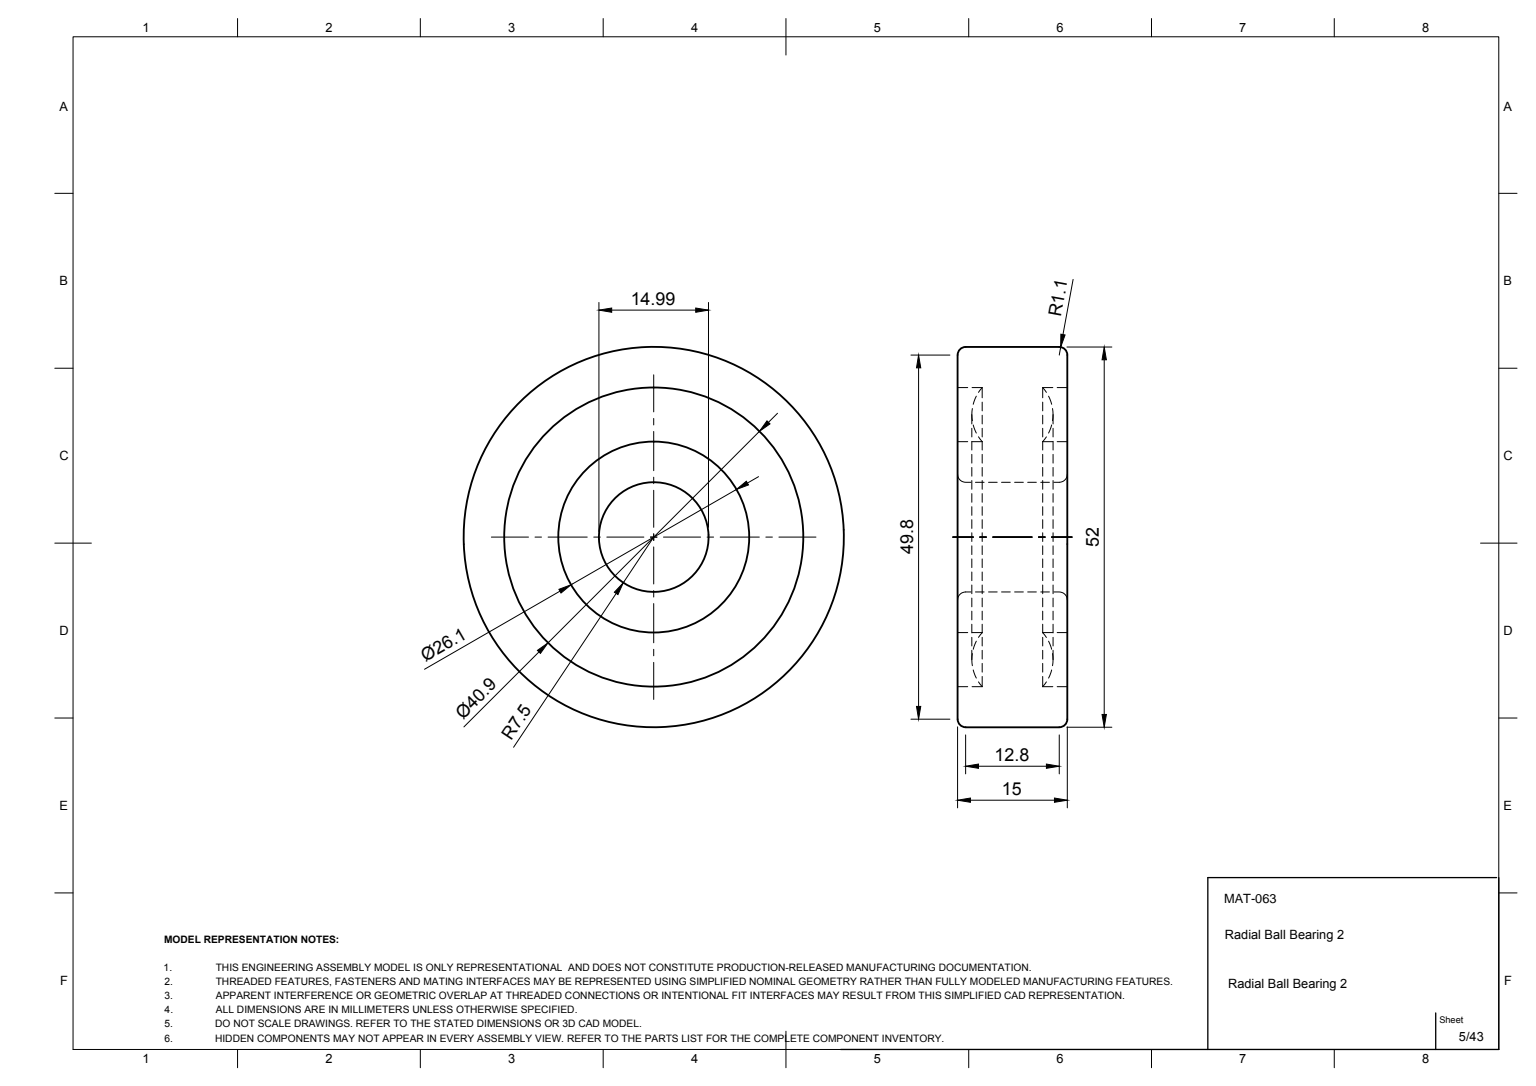
ISO-10303-21;
HEADER;
/* Generated by software containing ST-Developer
 * from STEP Tools, Inc. (www.steptools.com) 
 */

FILE_DESCRIPTION(
/* description */ (''),
/* implementation_level */ '2;1');

FILE_NAME(
/* name */ 'Radial Ball Bearing 2.step',
/* time_stamp */ '2026-10-24T09:43:01-07:00',
/* author */ (''),
/* organization */ (''),
/* preprocessor_version */ 'ST-DEVELOPER v20.2',
/* originating_system */ 'Autodesk Translation Framework v15.15.0.0',
/* authorisation */ '');

FILE_SCHEMA (('AUTOMOTIVE_DESIGN { 1 0 10303 214 3 1 1 }'));
ENDSEC;

DATA;
#10=MECHANICAL_DESIGN_GEOMETRIC_PRESENTATION_REPRESENTATION('',(#275),#11112);
#177=TOROIDAL_SURFACE('',#6521,0.0248999989285722,0.00110000131901909);
#178=TOROIDAL_SURFACE('',#6526,0.0248999989285722,0.00110000131901909);
#179=TOROIDAL_SURFACE('',#6534,0.0248999989285722,0.00110000131901911);
#180=TOROIDAL_SURFACE('',#6541,0.0248999989285722,0.00110000131901911);
#181=TOROIDAL_SURFACE('',#6545,0.01675,0.00555000054498457);
#182=TOROIDAL_SURFACE('',#6554,0.01675,0.00555000054498457);
#183=TOROIDAL_SURFACE('',#6563,0.00860000107142784,0.00110000131901912);
#184=TOROIDAL_SURFACE('',#6567,0.00860000107142784,0.00110000131901912);
#185=TOROIDAL_SURFACE('',#6575,0.00860000107142785,0.00110000131901912);
#186=TOROIDAL_SURFACE('',#6578,0.00860000107142785,0.00110000131901912);
#209=SHAPE_REPRESENTATION_RELATIONSHIP('SRR','None',#11232,#242);
#242=ADVANCED_BREP_SHAPE_REPRESENTATION('',(#308),#11077);
#275=STYLED_ITEM('',(#11425),#308);
#308=MANIFOLD_SOLID_BREP('Radial Ball Bearing 2',#6012);
#361=FACE_BOUND('',#1105,.T.);
#362=FACE_BOUND('',#1110,.T.);
#363=FACE_BOUND('',#1116,.T.);
#364=FACE_BOUND('',#1121,.T.);
#506=PLANE('',#6532);
#507=PLANE('',#6543);
#508=PLANE('',#6558);
#509=PLANE('',#6569);
#715=FACE_OUTER_BOUND('',#1101,.T.);
#716=FACE_OUTER_BOUND('',#1102,.T.);
#717=FACE_OUTER_BOUND('',#1103,.T.);
#718=FACE_OUTER_BOUND('',#1104,.T.);
#719=FACE_OUTER_BOUND('',#1106,.T.);
#720=FACE_OUTER_BOUND('',#1107,.T.);
#721=FACE_OUTER_BOUND('',#1108,.T.);
#722=FACE_OUTER_BOUND('',#1109,.T.);
#723=FACE_OUTER_BOUND('',#1111,.T.);
#724=FACE_OUTER_BOUND('',#1112,.T.);
#725=FACE_OUTER_BOUND('',#1113,.T.);
#726=FACE_OUTER_BOUND('',#1114,.T.);
#727=FACE_OUTER_BOUND('',#1115,.T.);
#728=FACE_OUTER_BOUND('',#1117,.T.);
#729=FACE_OUTER_BOUND('',#1118,.T.);
#730=FACE_OUTER_BOUND('',#1119,.T.);
#731=FACE_OUTER_BOUND('',#1120,.T.);
#732=FACE_OUTER_BOUND('',#1122,.T.);
#733=FACE_OUTER_BOUND('',#1123,.T.);
#734=FACE_OUTER_BOUND('',#1124,.T.);
#1101=EDGE_LOOP('',(#4133,#4134,#4135,#4136));
#1102=EDGE_LOOP('',(#4137,#4138,#4139,#4140));
#1103=EDGE_LOOP('',(#4141,#4142,#4143,#4144,#4145,#4146));
#1104=EDGE_LOOP('',(#4147,#4148));
#1105=EDGE_LOOP('',(#4149));
#1106=EDGE_LOOP('',(#4150,#4151,#4152,#4153));
#1107=EDGE_LOOP('',(#4154,#4155,#4156,#4157,#4158));
#1108=EDGE_LOOP('',(#4159,#4160,#4161,#4162));
#1109=EDGE_LOOP('',(#4163,#4164));
#1110=EDGE_LOOP('',(#4165));
#1111=EDGE_LOOP('',(#4166,#4167,#4168,#4169,#4170,#4171));
#1112=EDGE_LOOP('',(#4172,#4173,#4174,#4175,#4176));
#1113=EDGE_LOOP('',(#4177,#4178,#4179,#4180,#4181));
#1114=EDGE_LOOP('',(#4182,#4183,#4184,#4185,#4186,#4187));
#1115=EDGE_LOOP('',(#4188));
#1116=EDGE_LOOP('',(#4189,#4190));
#1117=EDGE_LOOP('',(#4191,#4192,#4193,#4194,#4195));
#1118=EDGE_LOOP('',(#4196,#4197,#4198,#4199));
#1119=EDGE_LOOP('',(#4200,#4201,#4202,#4203));
#1120=EDGE_LOOP('',(#4204));
#1121=EDGE_LOOP('',(#4205,#4206));
#1122=EDGE_LOOP('',(#4207,#4208,#4209,#4210,#4211,#4212));
#1123=EDGE_LOOP('',(#4213,#4214,#4215,#4216));
#1124=EDGE_LOOP('',(#4217,#4218,#4219,#4220));
#1580=LINE('',#9536,#1939);
#1581=LINE('',#9548,#1940);
#1582=LINE('',#9568,#1941);
#1583=LINE('',#9571,#1942);
#1584=LINE('',#9587,#1943);
#1585=LINE('',#9603,#1944);
#1939=VECTOR('',#7532,0.026);
#1940=VECTOR('',#7547,0.02045);
#1941=VECTOR('',#7574,0.02045);
#1942=VECTOR('',#7577,0.01305);
#1943=VECTOR('',#7598,0.01305);
#1944=VECTOR('',#7619,0.0075);
#2344=CIRCLE('',#6522,0.0248999997701383);
#2345=CIRCLE('',#6523,0.00110000131901909);
#2346=CIRCLE('',#6524,0.0260000002475909);
#2347=CIRCLE('',#6525,0.00110000131901909);
#2348=CIRCLE('',#6527,0.0248999997701383);
#2349=CIRCLE('',#6528,0.0260000002475909);
#2350=CIRCLE('',#6530,0.026);
#2351=CIRCLE('',#6531,0.026);
#2352=CIRCLE('',#6533,0.02045);
#2353=CIRCLE('',#6535,0.00110000131901911);
#2354=CIRCLE('',#6536,0.0248999997701383);
#2355=CIRCLE('',#6537,0.0011000013190191);
#2356=CIRCLE('',#6539,0.02045);
#2357=CIRCLE('',#6540,0.02045);
#2358=CIRCLE('',#6542,0.0248999997701383);
#2359=CIRCLE('',#6544,0.02045);
#2360=CIRCLE('',#6546,0.00555000054498457);
#2361=CIRCLE('',#6547,0.0130499999271107);
#2362=CIRCLE('',#6548,0.0130499999271107);
#2363=CIRCLE('',#6550,0.02045);
#2364=CIRCLE('',#6551,0.02045);
#2365=CIRCLE('',#6553,0.01305);
#2366=CIRCLE('',#6555,0.01305);
#2367=CIRCLE('',#6556,0.00555000054498457);
#2368=CIRCLE('',#6557,0.01305);
#2369=CIRCLE('',#6559,0.00860000022986177);
#2370=CIRCLE('',#6560,0.00860000022986177);
#2371=CIRCLE('',#6562,0.01305);
#2372=CIRCLE('',#6564,0.00110000131901912);
#2373=CIRCLE('',#6565,0.00749999975240907);
#2374=CIRCLE('',#6566,0.00110000131901912);
#2375=CIRCLE('',#6568,0.00749999975240873);
#2376=CIRCLE('',#6570,0.00860000022986177);
#2377=CIRCLE('',#6571,0.00860000022986177);
#2378=CIRCLE('',#6573,0.0075);
#2379=CIRCLE('',#6574,0.00749999975240873);
#2380=CIRCLE('',#6576,0.00110000131901912);
#2381=CIRCLE('',#6577,0.00110000131901912);
#2740=VERTEX_POINT('',#9520);
#2741=VERTEX_POINT('',#9521);
#2742=VERTEX_POINT('',#9523);
#2743=VERTEX_POINT('',#9525);
#2744=VERTEX_POINT('',#9532);
#2745=VERTEX_POINT('',#9533);
#2746=VERTEX_POINT('',#9538);
#2747=VERTEX_POINT('',#9541);
#2748=VERTEX_POINT('',#9543);
#2749=VERTEX_POINT('',#9547);
#2750=VERTEX_POINT('',#9549);
#2751=VERTEX_POINT('',#9555);
#2752=VERTEX_POINT('',#9558);
#2753=VERTEX_POINT('',#9560);
#2754=VERTEX_POINT('',#9564);
#2755=VERTEX_POINT('',#9565);
#2756=VERTEX_POINT('',#9570);
#2757=VERTEX_POINT('',#9574);
#2758=VERTEX_POINT('',#9575);
#2759=VERTEX_POINT('',#9580);
#2760=VERTEX_POINT('',#9581);
#2761=VERTEX_POINT('',#9585);
#2762=VERTEX_POINT('',#9589);
#2763=VERTEX_POINT('',#9591);
#2764=VERTEX_POINT('',#9597);
#2765=VERTEX_POINT('',#9598);
#2766=VERTEX_POINT('',#9602);
#2767=VERTEX_POINT('',#9604);
#3270=EDGE_CURVE('',#2740,#2741,#2344,.T.);
#3271=EDGE_CURVE('',#2741,#2742,#2345,.T.);
#3272=EDGE_CURVE('',#2742,#2743,#2346,.F.);
#3273=EDGE_CURVE('',#2743,#2740,#2347,.T.);
#3274=EDGE_CURVE('',#2741,#2740,#2348,.T.);
#3275=EDGE_CURVE('',#2743,#2742,#2349,.T.);
#3276=EDGE_CURVE('',#2744,#2745,#2350,.F.);
#3277=EDGE_CURVE('',#2745,#2744,#2351,.F.);
#3278=EDGE_CURVE('',#2744,#2742,#1580,.T.);
#3279=EDGE_CURVE('',#2746,#2746,#2352,.T.);
#3280=EDGE_CURVE('',#2744,#2747,#2353,.T.);
#3281=EDGE_CURVE('',#2747,#2748,#2354,.F.);
#3282=EDGE_CURVE('',#2748,#2745,#2355,.T.);
#3283=EDGE_CURVE('',#2746,#2749,#1581,.T.);
#3284=EDGE_CURVE('',#2750,#2749,#2356,.F.);
#3285=EDGE_CURVE('',#2749,#2750,#2357,.F.);
#3286=EDGE_CURVE('',#2748,#2747,#2358,.F.);
#3287=EDGE_CURVE('',#2751,#2751,#2359,.F.);
#3288=EDGE_CURVE('',#2750,#2752,#2360,.T.);
#3289=EDGE_CURVE('',#2752,#2753,#2361,.T.);
#3290=EDGE_CURVE('',#2753,#2752,#2362,.T.);
#3291=EDGE_CURVE('',#2754,#2755,#2363,.F.);
#3292=EDGE_CURVE('',#2755,#2754,#2364,.F.);
#3293=EDGE_CURVE('',#2755,#2751,#1582,.T.);
#3294=EDGE_CURVE('',#2753,#2756,#1583,.T.);
#3295=EDGE_CURVE('',#2756,#2756,#2365,.T.);
#3296=EDGE_CURVE('',#2757,#2758,#2366,.T.);
#3297=EDGE_CURVE('',#2758,#2754,#2367,.T.);
#3298=EDGE_CURVE('',#2758,#2757,#2368,.T.);
#3299=EDGE_CURVE('',#2759,#2760,#2369,.T.);
#3300=EDGE_CURVE('',#2760,#2759,#2370,.T.);
#3301=EDGE_CURVE('',#2761,#2761,#2371,.F.);
#3302=EDGE_CURVE('',#2761,#2757,#1584,.T.);
#3303=EDGE_CURVE('',#2760,#2762,#2372,.T.);
#3304=EDGE_CURVE('',#2762,#2763,#2373,.T.);
#3305=EDGE_CURVE('',#2763,#2759,#2374,.T.);
#3306=EDGE_CURVE('',#2763,#2762,#2375,.T.);
#3307=EDGE_CURVE('',#2764,#2765,#2376,.F.);
#3308=EDGE_CURVE('',#2765,#2764,#2377,.F.);
#3309=EDGE_CURVE('',#2762,#2766,#1585,.T.);
#3310=EDGE_CURVE('',#2767,#2766,#2378,.F.);
#3311=EDGE_CURVE('',#2766,#2767,#2379,.F.);
#3312=EDGE_CURVE('',#2766,#2764,#2380,.T.);
#3313=EDGE_CURVE('',#2765,#2767,#2381,.T.);
#4133=ORIENTED_EDGE('',*,*,#3270,.T.);
#4134=ORIENTED_EDGE('',*,*,#3271,.T.);
#4135=ORIENTED_EDGE('',*,*,#3272,.T.);
#4136=ORIENTED_EDGE('',*,*,#3273,.T.);
#4137=ORIENTED_EDGE('',*,*,#3271,.F.);
#4138=ORIENTED_EDGE('',*,*,#3274,.T.);
#4139=ORIENTED_EDGE('',*,*,#3273,.F.);
#4140=ORIENTED_EDGE('',*,*,#3275,.T.);
#4141=ORIENTED_EDGE('',*,*,#3276,.T.);
#4142=ORIENTED_EDGE('',*,*,#3277,.T.);
#4143=ORIENTED_EDGE('',*,*,#3278,.T.);
#4144=ORIENTED_EDGE('',*,*,#3275,.F.);
#4145=ORIENTED_EDGE('',*,*,#3272,.F.);
#4146=ORIENTED_EDGE('',*,*,#3278,.F.);
#4147=ORIENTED_EDGE('',*,*,#3270,.F.);
#4148=ORIENTED_EDGE('',*,*,#3274,.F.);
#4149=ORIENTED_EDGE('',*,*,#3279,.T.);
#4150=ORIENTED_EDGE('',*,*,#3276,.F.);
#4151=ORIENTED_EDGE('',*,*,#3280,.T.);
#4152=ORIENTED_EDGE('',*,*,#3281,.T.);
#4153=ORIENTED_EDGE('',*,*,#3282,.T.);
#4154=ORIENTED_EDGE('',*,*,#3279,.F.);
#4155=ORIENTED_EDGE('',*,*,#3283,.T.);
#4156=ORIENTED_EDGE('',*,*,#3284,.F.);
#4157=ORIENTED_EDGE('',*,*,#3285,.F.);
#4158=ORIENTED_EDGE('',*,*,#3283,.F.);
#4159=ORIENTED_EDGE('',*,*,#3280,.F.);
#4160=ORIENTED_EDGE('',*,*,#3277,.F.);
#4161=ORIENTED_EDGE('',*,*,#3282,.F.);
#4162=ORIENTED_EDGE('',*,*,#3286,.T.);
#4163=ORIENTED_EDGE('',*,*,#3281,.F.);
#4164=ORIENTED_EDGE('',*,*,#3286,.F.);
#4165=ORIENTED_EDGE('',*,*,#3287,.T.);
#4166=ORIENTED_EDGE('',*,*,#3285,.T.);
#4167=ORIENTED_EDGE('',*,*,#3288,.T.);
#4168=ORIENTED_EDGE('',*,*,#3289,.T.);
#4169=ORIENTED_EDGE('',*,*,#3290,.T.);
#4170=ORIENTED_EDGE('',*,*,#3288,.F.);
#4171=ORIENTED_EDGE('',*,*,#3284,.T.);
#4172=ORIENTED_EDGE('',*,*,#3291,.F.);
#4173=ORIENTED_EDGE('',*,*,#3292,.F.);
#4174=ORIENTED_EDGE('',*,*,#3293,.T.);
#4175=ORIENTED_EDGE('',*,*,#3287,.F.);
#4176=ORIENTED_EDGE('',*,*,#3293,.F.);
#4177=ORIENTED_EDGE('',*,*,#3290,.F.);
#4178=ORIENTED_EDGE('',*,*,#3294,.T.);
#4179=ORIENTED_EDGE('',*,*,#3295,.T.);
#4180=ORIENTED_EDGE('',*,*,#3294,.F.);
#4181=ORIENTED_EDGE('',*,*,#3289,.F.);
#4182=ORIENTED_EDGE('',*,*,#3296,.T.);
#4183=ORIENTED_EDGE('',*,*,#3297,.T.);
#4184=ORIENTED_EDGE('',*,*,#3291,.T.);
#4185=ORIENTED_EDGE('',*,*,#3292,.T.);
#4186=ORIENTED_EDGE('',*,*,#3297,.F.);
#4187=ORIENTED_EDGE('',*,*,#3298,.T.);
#4188=ORIENTED_EDGE('',*,*,#3295,.F.);
#4189=ORIENTED_EDGE('',*,*,#3299,.T.);
#4190=ORIENTED_EDGE('',*,*,#3300,.T.);
#4191=ORIENTED_EDGE('',*,*,#3301,.T.);
#4192=ORIENTED_EDGE('',*,*,#3302,.T.);
#4193=ORIENTED_EDGE('',*,*,#3298,.F.);
#4194=ORIENTED_EDGE('',*,*,#3296,.F.);
#4195=ORIENTED_EDGE('',*,*,#3302,.F.);
#4196=ORIENTED_EDGE('',*,*,#3303,.T.);
#4197=ORIENTED_EDGE('',*,*,#3304,.T.);
#4198=ORIENTED_EDGE('',*,*,#3305,.T.);
#4199=ORIENTED_EDGE('',*,*,#3300,.F.);
#4200=ORIENTED_EDGE('',*,*,#3306,.T.);
#4201=ORIENTED_EDGE('',*,*,#3303,.F.);
#4202=ORIENTED_EDGE('',*,*,#3299,.F.);
#4203=ORIENTED_EDGE('',*,*,#3305,.F.);
#4204=ORIENTED_EDGE('',*,*,#3301,.F.);
#4205=ORIENTED_EDGE('',*,*,#3307,.T.);
#4206=ORIENTED_EDGE('',*,*,#3308,.T.);
#4207=ORIENTED_EDGE('',*,*,#3304,.F.);
#4208=ORIENTED_EDGE('',*,*,#3309,.T.);
#4209=ORIENTED_EDGE('',*,*,#3310,.F.);
#4210=ORIENTED_EDGE('',*,*,#3311,.F.);
#4211=ORIENTED_EDGE('',*,*,#3309,.F.);
#4212=ORIENTED_EDGE('',*,*,#3306,.F.);
#4213=ORIENTED_EDGE('',*,*,#3312,.T.);
#4214=ORIENTED_EDGE('',*,*,#3308,.F.);
#4215=ORIENTED_EDGE('',*,*,#3313,.T.);
#4216=ORIENTED_EDGE('',*,*,#3310,.T.);
#4217=ORIENTED_EDGE('',*,*,#3307,.F.);
#4218=ORIENTED_EDGE('',*,*,#3312,.F.);
#4219=ORIENTED_EDGE('',*,*,#3311,.T.);
#4220=ORIENTED_EDGE('',*,*,#3313,.F.);
#5519=CYLINDRICAL_SURFACE('',#6529,0.026);
#5520=CYLINDRICAL_SURFACE('',#6538,0.02045);
#5521=CYLINDRICAL_SURFACE('',#6549,0.02045);
#5522=CYLINDRICAL_SURFACE('',#6552,0.01305);
#5523=CYLINDRICAL_SURFACE('',#6561,0.01305);
#5524=CYLINDRICAL_SURFACE('',#6572,0.0075);
#5688=ADVANCED_FACE('',(#715),#177,.T.);
#5689=ADVANCED_FACE('',(#716),#178,.T.);
#5690=ADVANCED_FACE('',(#717),#5519,.T.);
#5691=ADVANCED_FACE('',(#718,#361),#506,.T.);
#5692=ADVANCED_FACE('',(#719),#179,.T.);
#5693=ADVANCED_FACE('',(#720),#5520,.F.);
#5694=ADVANCED_FACE('',(#721),#180,.T.);
#5695=ADVANCED_FACE('',(#722,#362),#507,.T.);
#5696=ADVANCED_FACE('',(#723),#181,.T.);
#5697=ADVANCED_FACE('',(#724),#5521,.F.);
#5698=ADVANCED_FACE('',(#725),#5522,.T.);
#5699=ADVANCED_FACE('',(#726),#182,.T.);
#5700=ADVANCED_FACE('',(#727,#363),#508,.T.);
#5701=ADVANCED_FACE('',(#728),#5523,.T.);
#5702=ADVANCED_FACE('',(#729),#183,.T.);
#5703=ADVANCED_FACE('',(#730),#184,.T.);
#5704=ADVANCED_FACE('',(#731,#364),#509,.T.);
#5705=ADVANCED_FACE('',(#732),#5524,.F.);
#5706=ADVANCED_FACE('',(#733),#185,.T.);
#5707=ADVANCED_FACE('',(#734),#186,.T.);
#6012=CLOSED_SHELL('',(#5688,#5689,#5690,#5691,#5692,#5693,#5694,#5695,
#5696,#5697,#5698,#5699,#5700,#5701,#5702,#5703,#5704,#5705,#5706,#5707));
#6520=AXIS2_PLACEMENT_3D('',#9518,#7508,#7509);
#6521=AXIS2_PLACEMENT_3D('',#9519,#7510,#7511);
#6522=AXIS2_PLACEMENT_3D('',#9522,#7512,#7513);
#6523=AXIS2_PLACEMENT_3D('',#9524,#7514,#7515);
#6524=AXIS2_PLACEMENT_3D('',#9526,#7516,#7517);
#6525=AXIS2_PLACEMENT_3D('',#9527,#7518,#7519);
#6526=AXIS2_PLACEMENT_3D('',#9528,#7520,#7521);
#6527=AXIS2_PLACEMENT_3D('',#9529,#7522,#7523);
#6528=AXIS2_PLACEMENT_3D('',#9530,#7524,#7525);
#6529=AXIS2_PLACEMENT_3D('',#9531,#7526,#7527);
#6530=AXIS2_PLACEMENT_3D('',#9534,#7528,#7529);
#6531=AXIS2_PLACEMENT_3D('',#9535,#7530,#7531);
#6532=AXIS2_PLACEMENT_3D('',#9537,#7533,#7534);
#6533=AXIS2_PLACEMENT_3D('',#9539,#7535,#7536);
#6534=AXIS2_PLACEMENT_3D('',#9540,#7537,#7538);
#6535=AXIS2_PLACEMENT_3D('',#9542,#7539,#7540);
#6536=AXIS2_PLACEMENT_3D('',#9544,#7541,#7542);
#6537=AXIS2_PLACEMENT_3D('',#9545,#7543,#7544);
#6538=AXIS2_PLACEMENT_3D('',#9546,#7545,#7546);
#6539=AXIS2_PLACEMENT_3D('',#9550,#7548,#7549);
#6540=AXIS2_PLACEMENT_3D('',#9551,#7550,#7551);
#6541=AXIS2_PLACEMENT_3D('',#9552,#7552,#7553);
#6542=AXIS2_PLACEMENT_3D('',#9553,#7554,#7555);
#6543=AXIS2_PLACEMENT_3D('',#9554,#7556,#7557);
#6544=AXIS2_PLACEMENT_3D('',#9556,#7558,#7559);
#6545=AXIS2_PLACEMENT_3D('',#9557,#7560,#7561);
#6546=AXIS2_PLACEMENT_3D('',#9559,#7562,#7563);
#6547=AXIS2_PLACEMENT_3D('',#9561,#7564,#7565);
#6548=AXIS2_PLACEMENT_3D('',#9562,#7566,#7567);
#6549=AXIS2_PLACEMENT_3D('',#9563,#7568,#7569);
#6550=AXIS2_PLACEMENT_3D('',#9566,#7570,#7571);
#6551=AXIS2_PLACEMENT_3D('',#9567,#7572,#7573);
#6552=AXIS2_PLACEMENT_3D('',#9569,#7575,#7576);
#6553=AXIS2_PLACEMENT_3D('',#9572,#7578,#7579);
#6554=AXIS2_PLACEMENT_3D('',#9573,#7580,#7581);
#6555=AXIS2_PLACEMENT_3D('',#9576,#7582,#7583);
#6556=AXIS2_PLACEMENT_3D('',#9577,#7584,#7585);
#6557=AXIS2_PLACEMENT_3D('',#9578,#7586,#7587);
#6558=AXIS2_PLACEMENT_3D('',#9579,#7588,#7589);
#6559=AXIS2_PLACEMENT_3D('',#9582,#7590,#7591);
#6560=AXIS2_PLACEMENT_3D('',#9583,#7592,#7593);
#6561=AXIS2_PLACEMENT_3D('',#9584,#7594,#7595);
#6562=AXIS2_PLACEMENT_3D('',#9586,#7596,#7597);
#6563=AXIS2_PLACEMENT_3D('',#9588,#7599,#7600);
#6564=AXIS2_PLACEMENT_3D('',#9590,#7601,#7602);
#6565=AXIS2_PLACEMENT_3D('',#9592,#7603,#7604);
#6566=AXIS2_PLACEMENT_3D('',#9593,#7605,#7606);
#6567=AXIS2_PLACEMENT_3D('',#9594,#7607,#7608);
#6568=AXIS2_PLACEMENT_3D('',#9595,#7609,#7610);
#6569=AXIS2_PLACEMENT_3D('',#9596,#7611,#7612);
#6570=AXIS2_PLACEMENT_3D('',#9599,#7613,#7614);
#6571=AXIS2_PLACEMENT_3D('',#9600,#7615,#7616);
#6572=AXIS2_PLACEMENT_3D('',#9601,#7617,#7618);
#6573=AXIS2_PLACEMENT_3D('',#9605,#7620,#7621);
#6574=AXIS2_PLACEMENT_3D('',#9606,#7622,#7623);
#6575=AXIS2_PLACEMENT_3D('',#9607,#7624,#7625);
#6576=AXIS2_PLACEMENT_3D('',#9608,#7626,#7627);
#6577=AXIS2_PLACEMENT_3D('',#9609,#7628,#7629);
#6578=AXIS2_PLACEMENT_3D('',#9610,#7630,#7631);
#7508=DIRECTION('axis',(0.,0.,1.));
#7509=DIRECTION('refdir',(1.,0.,0.));
#7510=DIRECTION('center_axis',(1.,4.17203717831812E-9,1.01277540341552E-17));
#7511=DIRECTION('ref_axis',(-4.1720371751696E-9,1.,0.));
#7512=DIRECTION('center_axis',(1.,4.17203717831812E-9,1.01277540341552E-17));
#7513=DIRECTION('ref_axis',(-4.17203717831812E-9,1.,-1.69634196247466E-42));
#7514=DIRECTION('center_axis',(8.36866394062756E-10,1.,-8.36884415538179E-10));
#7515=DIRECTION('ref_axis',(-7.96162761077703E-7,8.36885081819775E-10,0.999999999999683));
#7516=DIRECTION('center_axis',(1.,4.17203717831812E-9,1.01277540341552E-17));
#7517=DIRECTION('ref_axis',(-4.17203717831812E-9,1.,-1.69634196247466E-42));
#7518=DIRECTION('center_axis',(8.36869948186391E-10,1.,8.36891441629708E-10));
#7519=DIRECTION('ref_axis',(-0.999999999999707,8.36870588457614E-10,-7.65059166582913E-7));
#7520=DIRECTION('center_axis',(1.,-4.17203708245403E-9,6.73890284431642E-18));
#7521=DIRECTION('ref_axis',(-4.1720370750894E-9,-1.,5.66553889764798E-16));
#7522=DIRECTION('center_axis',(1.,-4.17203708245403E-9,6.73890284431642E-18));
#7523=DIRECTION('ref_axis',(4.17203708245403E-9,1.,-1.23465054354127E-43));
#7524=DIRECTION('center_axis',(-1.,4.17203697154146E-9,4.27849718847752E-19));
#7525=DIRECTION('ref_axis',(-4.27008851558771E-17,-5.34839554841822E-9,
1.));
#7526=DIRECTION('center_axis',(1.,0.,-3.33600668457079E-17));
#7527=DIRECTION('ref_axis',(-3.33600668457079E-17,0.,-1.));
#7528=DIRECTION('center_axis',(1.,0.,-3.33600668457079E-17));
#7529=DIRECTION('ref_axis',(-3.33600668457079E-17,0.,-1.));
#7530=DIRECTION('center_axis',(1.,0.,0.));
#7531=DIRECTION('ref_axis',(0.,-4.64793894161955E-10,-1.));
#7532=DIRECTION('',(-1.,0.,3.33600668457079E-17));
#7533=DIRECTION('center_axis',(-1.,1.53144334479515E-17,1.9842828066192E-17));
#7534=DIRECTION('ref_axis',(1.9842828066192E-17,0.,1.));
#7535=DIRECTION('center_axis',(1.,0.,0.));
#7536=DIRECTION('ref_axis',(0.,0.,-1.));
#7537=DIRECTION('center_axis',(1.,-4.17203727418451E-9,-1.07069540457721E-17));
#7538=DIRECTION('ref_axis',(4.1720372752498E-9,1.,0.));
#7539=DIRECTION('center_axis',(-8.36866342496331E-10,1.,-8.36883936494317E-10));
#7540=DIRECTION('ref_axis',(0.999999999999707,8.36866982761818E-10,7.65059174657239E-7));
#7541=DIRECTION('center_axis',(1.,-4.17203727418451E-9,-1.07069540457721E-17));
#7542=DIRECTION('ref_axis',(4.17203727418451E-9,1.,1.45967462857766E-42));
#7543=DIRECTION('center_axis',(-8.36844869453255E-10,1.,8.36865935422119E-10));
#7544=DIRECTION('ref_axis',(9.00645352209864E-7,8.36866689122222E-10,-0.999999999999595));
#7545=DIRECTION('center_axis',(1.,0.,0.));
#7546=DIRECTION('ref_axis',(0.,0.,-1.));
#7547=DIRECTION('',(1.,0.,0.));
#7548=DIRECTION('center_axis',(1.,0.,0.));
#7549=DIRECTION('ref_axis',(0.,-4.29586394988857E-10,-1.));
#7550=DIRECTION('center_axis',(1.,0.,0.));
#7551=DIRECTION('ref_axis',(0.,-4.29586394988857E-10,-1.));
#7552=DIRECTION('center_axis',(1.,4.17203725971588E-9,2.0031116033889E-18));
#7553=DIRECTION('ref_axis',(4.1720372752498E-9,-1.,5.66553889764798E-16));
#7554=DIRECTION('center_axis',(1.,4.17203725971588E-9,2.0031116033889E-18));
#7555=DIRECTION('ref_axis',(-4.17203725971588E-9,1.,5.39459847610519E-43));
#7556=DIRECTION('center_axis',(1.,1.53144334479515E-17,-1.9842828066192E-17));
#7557=DIRECTION('ref_axis',(-1.9842828066192E-17,0.,-1.));
#7558=DIRECTION('center_axis',(1.,0.,0.));
#7559=DIRECTION('ref_axis',(0.,0.,-1.));
#7560=DIRECTION('center_axis',(1.,6.36556116938371E-17,1.00386354793954E-17));
#7561=DIRECTION('ref_axis',(-6.3655612933414E-17,1.,0.));
#7562=DIRECTION('center_axis',(1.00386354793954E-17,1.22464679914735E-16,
-1.));
#7563=DIRECTION('ref_axis',(6.36556105223495E-17,-1.,-1.22464679914735E-16));
#7564=DIRECTION('center_axis',(1.,1.35504238326755E-16,2.34999225611352E-17));
#7565=DIRECTION('ref_axis',(-1.35504238326755E-16,1.,1.40763492406121E-49));
#7566=DIRECTION('center_axis',(1.,1.35504238326755E-16,2.34999225611352E-17));
#7567=DIRECTION('ref_axis',(-1.35504238326755E-16,1.,1.40763492406121E-49));
#7568=DIRECTION('center_axis',(1.,0.,0.));
#7569=DIRECTION('ref_axis',(0.,0.,-1.));
#7570=DIRECTION('center_axis',(-1.,0.,0.));
#7571=DIRECTION('ref_axis',(0.,-6.60206605267583E-10,1.));
#7572=DIRECTION('center_axis',(-1.,0.,0.));
#7573=DIRECTION('ref_axis',(0.,-6.60206605267583E-10,1.));
#7574=DIRECTION('',(1.,0.,0.));
#7575=DIRECTION('center_axis',(1.,0.,0.));
#7576=DIRECTION('ref_axis',(0.,0.,-1.));
#7577=DIRECTION('',(-1.,0.,0.));
#7578=DIRECTION('center_axis',(1.,0.,0.));
#7579=DIRECTION('ref_axis',(0.,0.,-1.));
#7580=DIRECTION('center_axis',(1.,1.18552772674719E-16,-1.97711088800387E-17));
#7581=DIRECTION('ref_axis',(-1.18552772074394E-16,1.,0.));
#7582=DIRECTION('center_axis',(-1.,0.,0.));
#7583=DIRECTION('ref_axis',(0.,-2.05103586755523E-10,1.));
#7584=DIRECTION('center_axis',(-1.97711088800387E-17,1.22464679914735E-16,
-1.));
#7585=DIRECTION('ref_axis',(1.18552771796194E-16,-1.,-1.22464679914735E-16));
#7586=DIRECTION('center_axis',(-1.,0.,0.));
#7587=DIRECTION('ref_axis',(0.,-2.05103586755523E-10,1.));
#7588=DIRECTION('center_axis',(-1.,2.92206431305708E-17,3.78610282642285E-17));
#7589=DIRECTION('ref_axis',(3.78610282642285E-17,0.,1.));
#7590=DIRECTION('center_axis',(1.,1.20795004338275E-8,6.525328094131E-17));
#7591=DIRECTION('ref_axis',(-1.20795004338275E-8,1.,4.44135209129409E-41));
#7592=DIRECTION('center_axis',(1.,-1.20794999078492E-8,-6.65136044666218E-17));
#7593=DIRECTION('ref_axis',(1.20794999078492E-8,1.,-3.20659696454606E-41));
#7594=DIRECTION('center_axis',(1.,0.,0.));
#7595=DIRECTION('ref_axis',(0.,0.,-1.));
#7596=DIRECTION('center_axis',(1.,0.,0.));
#7597=DIRECTION('ref_axis',(0.,0.,-1.));
#7598=DIRECTION('',(-1.,0.,0.));
#7599=DIRECTION('center_axis',(1.,-1.20794999078492E-8,-6.65136044666218E-17));
#7600=DIRECTION('ref_axis',(-1.20794999243885E-8,-1.,-5.21792575105832E-12));
#7601=DIRECTION('center_axis',(-3.90112644891662E-10,-1.,-3.90117034748036E-10));
#7602=DIRECTION('ref_axis',(-7.96162782272821E-7,3.90117345341081E-10,-0.999999999999683));
#7603=DIRECTION('center_axis',(1.,-1.20794992145421E-8,-4.8381018443521E-19));
#7604=DIRECTION('ref_axis',(1.48029741503464E-16,1.78300800621899E-8,-1.));
#7605=DIRECTION('center_axis',(-3.90083830404282E-10,-1.,3.90119162273478E-10));
#7606=DIRECTION('ref_axis',(-0.999999999999707,3.90084128868405E-10,7.65059156489968E-7));
#7607=DIRECTION('center_axis',(1.,1.20795004338275E-8,6.525328094131E-17));
#7608=DIRECTION('ref_axis',(-1.20795004609008E-8,1.,0.));
#7609=DIRECTION('center_axis',(1.,1.20795004338275E-8,6.525328094131E-17));
#7610=DIRECTION('ref_axis',(-1.20795004338275E-8,1.,4.44135209129409E-41));
#7611=DIRECTION('center_axis',(1.,2.92206431305708E-17,-3.78610282642285E-17));
#7612=DIRECTION('ref_axis',(-3.78610282642285E-17,0.,-1.));
#7613=DIRECTION('center_axis',(1.,-1.20794999071527E-8,2.28224857621035E-17));
#7614=DIRECTION('ref_axis',(1.20794999071527E-8,1.,-1.89856639006012E-41));
#7615=DIRECTION('center_axis',(1.,1.20794999172425E-8,-1.59545740616835E-17));
#7616=DIRECTION('ref_axis',(-1.20794999172425E-8,1.,2.99570552288603E-42));
#7617=DIRECTION('center_axis',(1.,0.,-1.15648231731787E-16));
#7618=DIRECTION('ref_axis',(-1.15648231731787E-16,0.,-1.));
#7619=DIRECTION('',(1.,0.,-1.15648231731787E-16));
#7620=DIRECTION('center_axis',(1.,0.,0.));
#7621=DIRECTION('ref_axis',(0.,-4.29586131949163E-10,-1.));
#7622=DIRECTION('center_axis',(1.,-1.20794999071527E-8,2.28224857621035E-17));
#7623=DIRECTION('ref_axis',(1.20794999071527E-8,1.,-1.89856639006012E-41));
#7624=DIRECTION('center_axis',(1.,1.20794999172425E-8,-1.59545740616835E-17));
#7625=DIRECTION('ref_axis',(1.20794999243885E-8,-1.,-8.2319592183107E-12));
#7626=DIRECTION('center_axis',(3.9010897446429E-10,-1.,-3.90108144056802E-10));
#7627=DIRECTION('ref_axis',(0.999999999999707,3.90109272919983E-10,-7.65059154471383E-7));
#7628=DIRECTION('center_axis',(3.90083837031876E-10,-1.,3.90119162425402E-10));
#7629=DIRECTION('ref_axis',(7.96162783282112E-7,3.90119472995512E-10,0.999999999999683));
#7630=DIRECTION('center_axis',(1.,-1.20794999071527E-8,2.28224857621035E-17));
#7631=DIRECTION('ref_axis',(1.20794999243885E-8,1.,0.));
#9518=CARTESIAN_POINT('',(0.,0.,0.));
#9519=CARTESIAN_POINT('Origin',(-0.00639999889435817,-1.33725586897056E-10,
-2.60202312123977E-18));
#9520=CARTESIAN_POINT('',(-0.00750000021337694,-2.62982038223811E-17,-0.0248999997701383));
#9521=CARTESIAN_POINT('',(-0.00750000021337694,-9.33158505355009E-18,0.0248999997701383));
#9522=CARTESIAN_POINT('Origin',(-0.00750000021337694,-1.38314833296201E-10,
-2.61316366403604E-18));
#9523=CARTESIAN_POINT('',(-0.00639999976976533,-1.58005919577827E-12,0.0260000002475909));
#9524=CARTESIAN_POINT('Origin',(-0.00639999889435817,-9.20581548326642E-13,
0.0248999989285722));
#9525=CARTESIAN_POINT('',(-0.00639999976976533,-3.35121902792442E-17,-0.0260000002475909));
#9526=CARTESIAN_POINT('Origin',(-0.00639999977013826,-1.33725590550843E-10,
-2.60202313010945E-18));
#9527=CARTESIAN_POINT('Origin',(-0.00639999889435817,-9.20629689158185E-13,
-0.0248999989285722));
#9528=CARTESIAN_POINT('Origin',(-0.00639999889435817,1.33725588194013E-10,
-2.25687613815873E-19));
#9529=CARTESIAN_POINT('Origin',(-0.00750000021337694,1.38314834487708E-10,
-2.3310041583336E-19));
#9530=CARTESIAN_POINT('Origin',(-0.00639999977013826,1.3372558821988E-10,
4.44089209850063E-18));
#9531=CARTESIAN_POINT('Origin',(-0.0206375,0.,-4.33144407778805E-52));
#9532=CARTESIAN_POINT('',(0.00639999998722997,-6.70342338705283E-12,0.0260000000825303));
#9533=CARTESIAN_POINT('',(0.00639999998722997,-5.37097589710219E-12,-0.0260000000825303));
#9534=CARTESIAN_POINT('Origin',(0.0064,0.,-9.01972807340825E-19));
#9535=CARTESIAN_POINT('Origin',(0.0064,2.91826343292479E-18,0.));
#9536=CARTESIAN_POINT('',(-0.0206375,-3.18408167778312E-18,0.026));
#9537=CARTESIAN_POINT('Origin',(-0.0075,-1.31838984174237E-18,-1.2490009027033E-18));
#9538=CARTESIAN_POINT('',(-0.0075,-2.50440270425634E-18,0.02045));
#9539=CARTESIAN_POINT('Origin',(-0.0075,0.,0.));
#9540=CARTESIAN_POINT('Origin',(0.00639999889435816,-1.33725593635445E-10,
-3.59711256079879E-19));
#9541=CARTESIAN_POINT('',(0.00750000021337694,-1.05191955076574E-17,0.0248999997701383));
#9542=CARTESIAN_POINT('Origin',(0.00639999889435816,-9.20588335445364E-13,
0.0248999989285722));
#9543=CARTESIAN_POINT('',(0.00750000021337694,-2.93287844693988E-17,-0.0248999997701383));
#9544=CARTESIAN_POINT('Origin',(0.00750000021337694,-1.38314840140043E-10,
-3.71488919652902E-19));
#9545=CARTESIAN_POINT('Origin',(0.00639999889435816,-9.20608946339399E-13,
-0.0248999989285722));
#9546=CARTESIAN_POINT('Origin',(-0.0206375,0.,0.));
#9547=CARTESIAN_POINT('',(-0.00413672599961696,1.0458235455062E-18,0.0204500000364447));
#9548=CARTESIAN_POINT('',(-0.0206375,-2.50440270425634E-18,0.02045));
#9549=CARTESIAN_POINT('',(-0.004136726,-0.02045,-2.79956704802153E-18));
#9550=CARTESIAN_POINT('Origin',(-0.004136726,1.15025496390116E-19,8.88178419700125E-18));
#9551=CARTESIAN_POINT('Origin',(-0.004136726,1.15025496390116E-19,8.88178419700125E-18));
#9552=CARTESIAN_POINT('Origin',(0.00639999889435816,1.33725592594967E-10,
2.43522299685913E-19));
#9553=CARTESIAN_POINT('Origin',(0.00750000021337694,1.3831483908365E-10,
2.45725725091783E-19));
#9554=CARTESIAN_POINT('Origin',(0.0075,-1.31838984174237E-18,1.2490009027033E-18));
#9555=CARTESIAN_POINT('',(0.0075,-2.50440270425634E-18,0.02045));
#9556=CARTESIAN_POINT('Origin',(0.0075,0.,0.));
#9557=CARTESIAN_POINT('Origin',(4.25120033285821E-10,2.32696931299848E-18,
-2.53637255105429E-19));
#9558=CARTESIAN_POINT('',(-0.00413672599923392,-0.0130499999271107,-1.89332840771843E-18));
#9559=CARTESIAN_POINT('Origin',(4.25120034352053E-10,-0.01675,-2.30492064367725E-18));
#9560=CARTESIAN_POINT('',(-0.00413672599923392,-9.72427111671565E-12,0.0130499999635554));
#9561=CARTESIAN_POINT('Origin',(-0.00413672599923392,-2.48296911984889E-18,
-8.56610574398074E-20));
#9562=CARTESIAN_POINT('Origin',(-0.00413672599923392,-2.48296911984889E-18,
-8.56610574398074E-20));
#9563=CARTESIAN_POINT('Origin',(-0.0206375,0.,0.));
#9564=CARTESIAN_POINT('',(0.004136726,-0.02045,-1.97855791081413E-18));
#9565=CARTESIAN_POINT('',(0.004136726,-2.50440270425634E-18,0.02045));
#9566=CARTESIAN_POINT('Origin',(0.004136726,-1.49874617044541E-18,-8.88178419700125E-18));
#9567=CARTESIAN_POINT('Origin',(0.004136726,-1.49874617044541E-18,-8.88178419700125E-18));
#9568=CARTESIAN_POINT('',(-0.0206375,-2.50440270425634E-18,0.02045));
#9569=CARTESIAN_POINT('Origin',(-0.0206375,0.,0.));
#9570=CARTESIAN_POINT('',(-0.0075,-1.5981640728873E-18,0.01305));
#9571=CARTESIAN_POINT('',(-0.0206375,-1.5981640728873E-18,0.01305));
#9572=CARTESIAN_POINT('Origin',(-0.0075,0.,0.));
#9573=CARTESIAN_POINT('Origin',(-4.25120036303284E-10,3.75386134271222E-18,
6.07632462000188E-19));
#9574=CARTESIAN_POINT('',(0.00413672599923392,-2.67659699192252E-12,0.0130499999635553));
#9575=CARTESIAN_POINT('',(0.00413672599923392,-0.01305,-1.07231927942994E-18));
#9576=CARTESIAN_POINT('Origin',(0.00413672599923392,-3.3221160294436E-19,
2.22044604925031E-18));
#9577=CARTESIAN_POINT('Origin',(-4.25120034317525E-10,-0.01675,-1.44365092657163E-18));
#9578=CARTESIAN_POINT('Origin',(0.00413672599923392,-3.3221160294436E-19,
2.22044604925031E-18));
#9579=CARTESIAN_POINT('Origin',(-0.0075,-1.3010426069826E-19,-1.1666015375944E-18));
#9580=CARTESIAN_POINT('',(-0.00750000021337695,-7.32444758467801E-18,-0.00860000022986174));
#9581=CARTESIAN_POINT('',(-0.00750000021337695,-9.55563692214474E-13,0.00860000022983698));
#9582=CARTESIAN_POINT('Origin',(-0.00750000021337695,1.20438122996688E-10,
1.91155415755433E-19));
#9583=CARTESIAN_POINT('Origin',(-0.00750000021337695,-1.20438124044286E-10,
-1.263242268E-19));
#9584=CARTESIAN_POINT('Origin',(-0.0206375,0.,0.));
#9585=CARTESIAN_POINT('',(0.0075,-1.5981640728873E-18,0.01305));
#9586=CARTESIAN_POINT('Origin',(0.0075,0.,0.));
#9587=CARTESIAN_POINT('',(-0.0206375,-1.5981640728873E-18,0.01305));
#9588=CARTESIAN_POINT('Origin',(-0.00639999889435815,-1.33725589876008E-10,
-1.99489279445979E-19));
#9589=CARTESIAN_POINT('',(-0.00639999933187528,-1.78004529143068E-13,0.00749999975240887));
#9590=CARTESIAN_POINT('Origin',(-0.00639999889435815,-4.29138899262724E-13,
0.00860000107142784));
#9591=CARTESIAN_POINT('',(-0.00639999933187528,7.82593383085413E-14,-0.00749999975240887));
#9592=CARTESIAN_POINT('Origin',(-0.00639999977013826,-1.33725577217623E-10,
-2.22044604925031E-18));
#9593=CARTESIAN_POINT('Origin',(-0.00639999889435815,-4.29112928832131E-13,
-0.00860000107142784));
#9594=CARTESIAN_POINT('Origin',(-0.00639999889435816,1.33725589406987E-10,
2.62934110861178E-19));
#9595=CARTESIAN_POINT('Origin',(-0.00639999889435816,1.33725589406987E-10,
2.62934110861178E-19));
#9596=CARTESIAN_POINT('Origin',(0.0075,-1.3010426069826E-19,1.1666015375944E-18));
#9597=CARTESIAN_POINT('',(0.00750000021337695,-1.12844211802569E-18,0.00860000022986174));
#9598=CARTESIAN_POINT('',(0.00750000021337695,-9.55567354576375E-13,-0.00860000022983698));
#9599=CARTESIAN_POINT('Origin',(0.00750000021337695,1.20438122943562E-10,
-1.36910420000699E-19));
#9600=CARTESIAN_POINT('Origin',(0.00750000021337695,-1.20438123513651E-10,
2.9038238015475E-19));
#9601=CARTESIAN_POINT('Origin',(-0.0206375,0.,-2.49552314011156E-51));
#9602=CARTESIAN_POINT('',(0.00639999944717908,-3.41326938021997E-12,0.00749999987620436));
#9603=CARTESIAN_POINT('',(-0.0206375,-9.18485099360515E-19,0.0075));
#9604=CARTESIAN_POINT('',(0.00639999944670613,1.23481356905966E-13,-0.0074999998349392));
#9605=CARTESIAN_POINT('Origin',(0.0064,-1.93061231994698E-18,-5.55111512312578E-18));
#9606=CARTESIAN_POINT('Origin',(0.00639999889435815,1.33725588774518E-10,
-1.62015184442301E-19));
#9607=CARTESIAN_POINT('Origin',(0.00639999889435815,-1.33725589355705E-10,
3.07932432666985E-19));
#9608=CARTESIAN_POINT('Origin',(0.00639999889435815,-4.29128599184298E-13,
0.00860000107142785));
#9609=CARTESIAN_POINT('Origin',(0.00639999889435815,-4.2911240869608E-13,
-0.00860000107142785));
#9610=CARTESIAN_POINT('Origin',(0.00639999889435815,1.33725588774518E-10,
-1.62015184442301E-19));
#11038=UNCERTAINTY_MEASURE_WITH_UNIT(LENGTH_MEASURE(1.E-5),#11113,
'DISTANCE_ACCURACY_VALUE',
'Maximum model space distance between geometric entities at asserted c
onnectivities');
#11073=UNCERTAINTY_MEASURE_WITH_UNIT(LENGTH_MEASURE(1.E-5),#11113,
'DISTANCE_ACCURACY_VALUE',
'Maximum model space distance between geometric entities at asserted c
onnectivities');
#11077=(
GEOMETRIC_REPRESENTATION_CONTEXT(3)
GLOBAL_UNCERTAINTY_ASSIGNED_CONTEXT((#11038))
GLOBAL_UNIT_ASSIGNED_CONTEXT((#11113,#11114,#11115))
REPRESENTATION_CONTEXT('','3D')
);
#11112=(
GEOMETRIC_REPRESENTATION_CONTEXT(3)
GLOBAL_UNCERTAINTY_ASSIGNED_CONTEXT((#11073))
GLOBAL_UNIT_ASSIGNED_CONTEXT((#11113,#11114,#11115))
REPRESENTATION_CONTEXT('','3D')
);
#11113=(
LENGTH_UNIT()
NAMED_UNIT(*)
SI_UNIT($,.METRE.)
);
#11114=(
NAMED_UNIT(*)
PLANE_ANGLE_UNIT()
SI_UNIT($,.RADIAN.)
);
#11115=(
NAMED_UNIT(*)
SI_UNIT($,.STERADIAN.)
SOLID_ANGLE_UNIT()
);
#11119=SHAPE_DEFINITION_REPRESENTATION(#11157,#11232);
#11157=PRODUCT_DEFINITION_SHAPE('',$,#11271);
#11232=SHAPE_REPRESENTATION('',(#6520),#11077);
#11267=PRODUCT_DEFINITION_CONTEXT('part definition',#11383,'design');
#11271=PRODUCT_DEFINITION('Radial Ball Bearing 2',
'Radial Ball Bearing 2',#11309,#11267);
#11309=PRODUCT_DEFINITION_FORMATION('',$,#11388);
#11383=APPLICATION_CONTEXT(
'Core Data for Automotive Mechanical Design Process');
#11384=PRODUCT_CONTEXT('part definition',#11383,'mechanical');
#11388=PRODUCT('Radial Ball Bearing 2','Radial Ball Bearing 2',
'radial ball bearing_68_as_AS_ISO 15 RBB - 415 - 6,SI,NC,6_68__ DE    
10847',(#11384));
#11425=PRESENTATION_STYLE_ASSIGNMENT((#11429));
#11429=SURFACE_STYLE_USAGE(.BOTH.,#11433);
#11433=SURFACE_SIDE_STYLE('',(#11437));
#11437=SURFACE_STYLE_FILL_AREA(#11441);
#11441=FILL_AREA_STYLE('Opaque(255,242,232)',(#11445));
#11445=FILL_AREA_STYLE_COLOUR('Opaque(255,242,232)',#11449);
#11449=COLOUR_RGB('Opaque(255,242,232)',1.,0.949019607843137,0.909803921568627);
ENDSEC;
END-ISO-10303-21;
